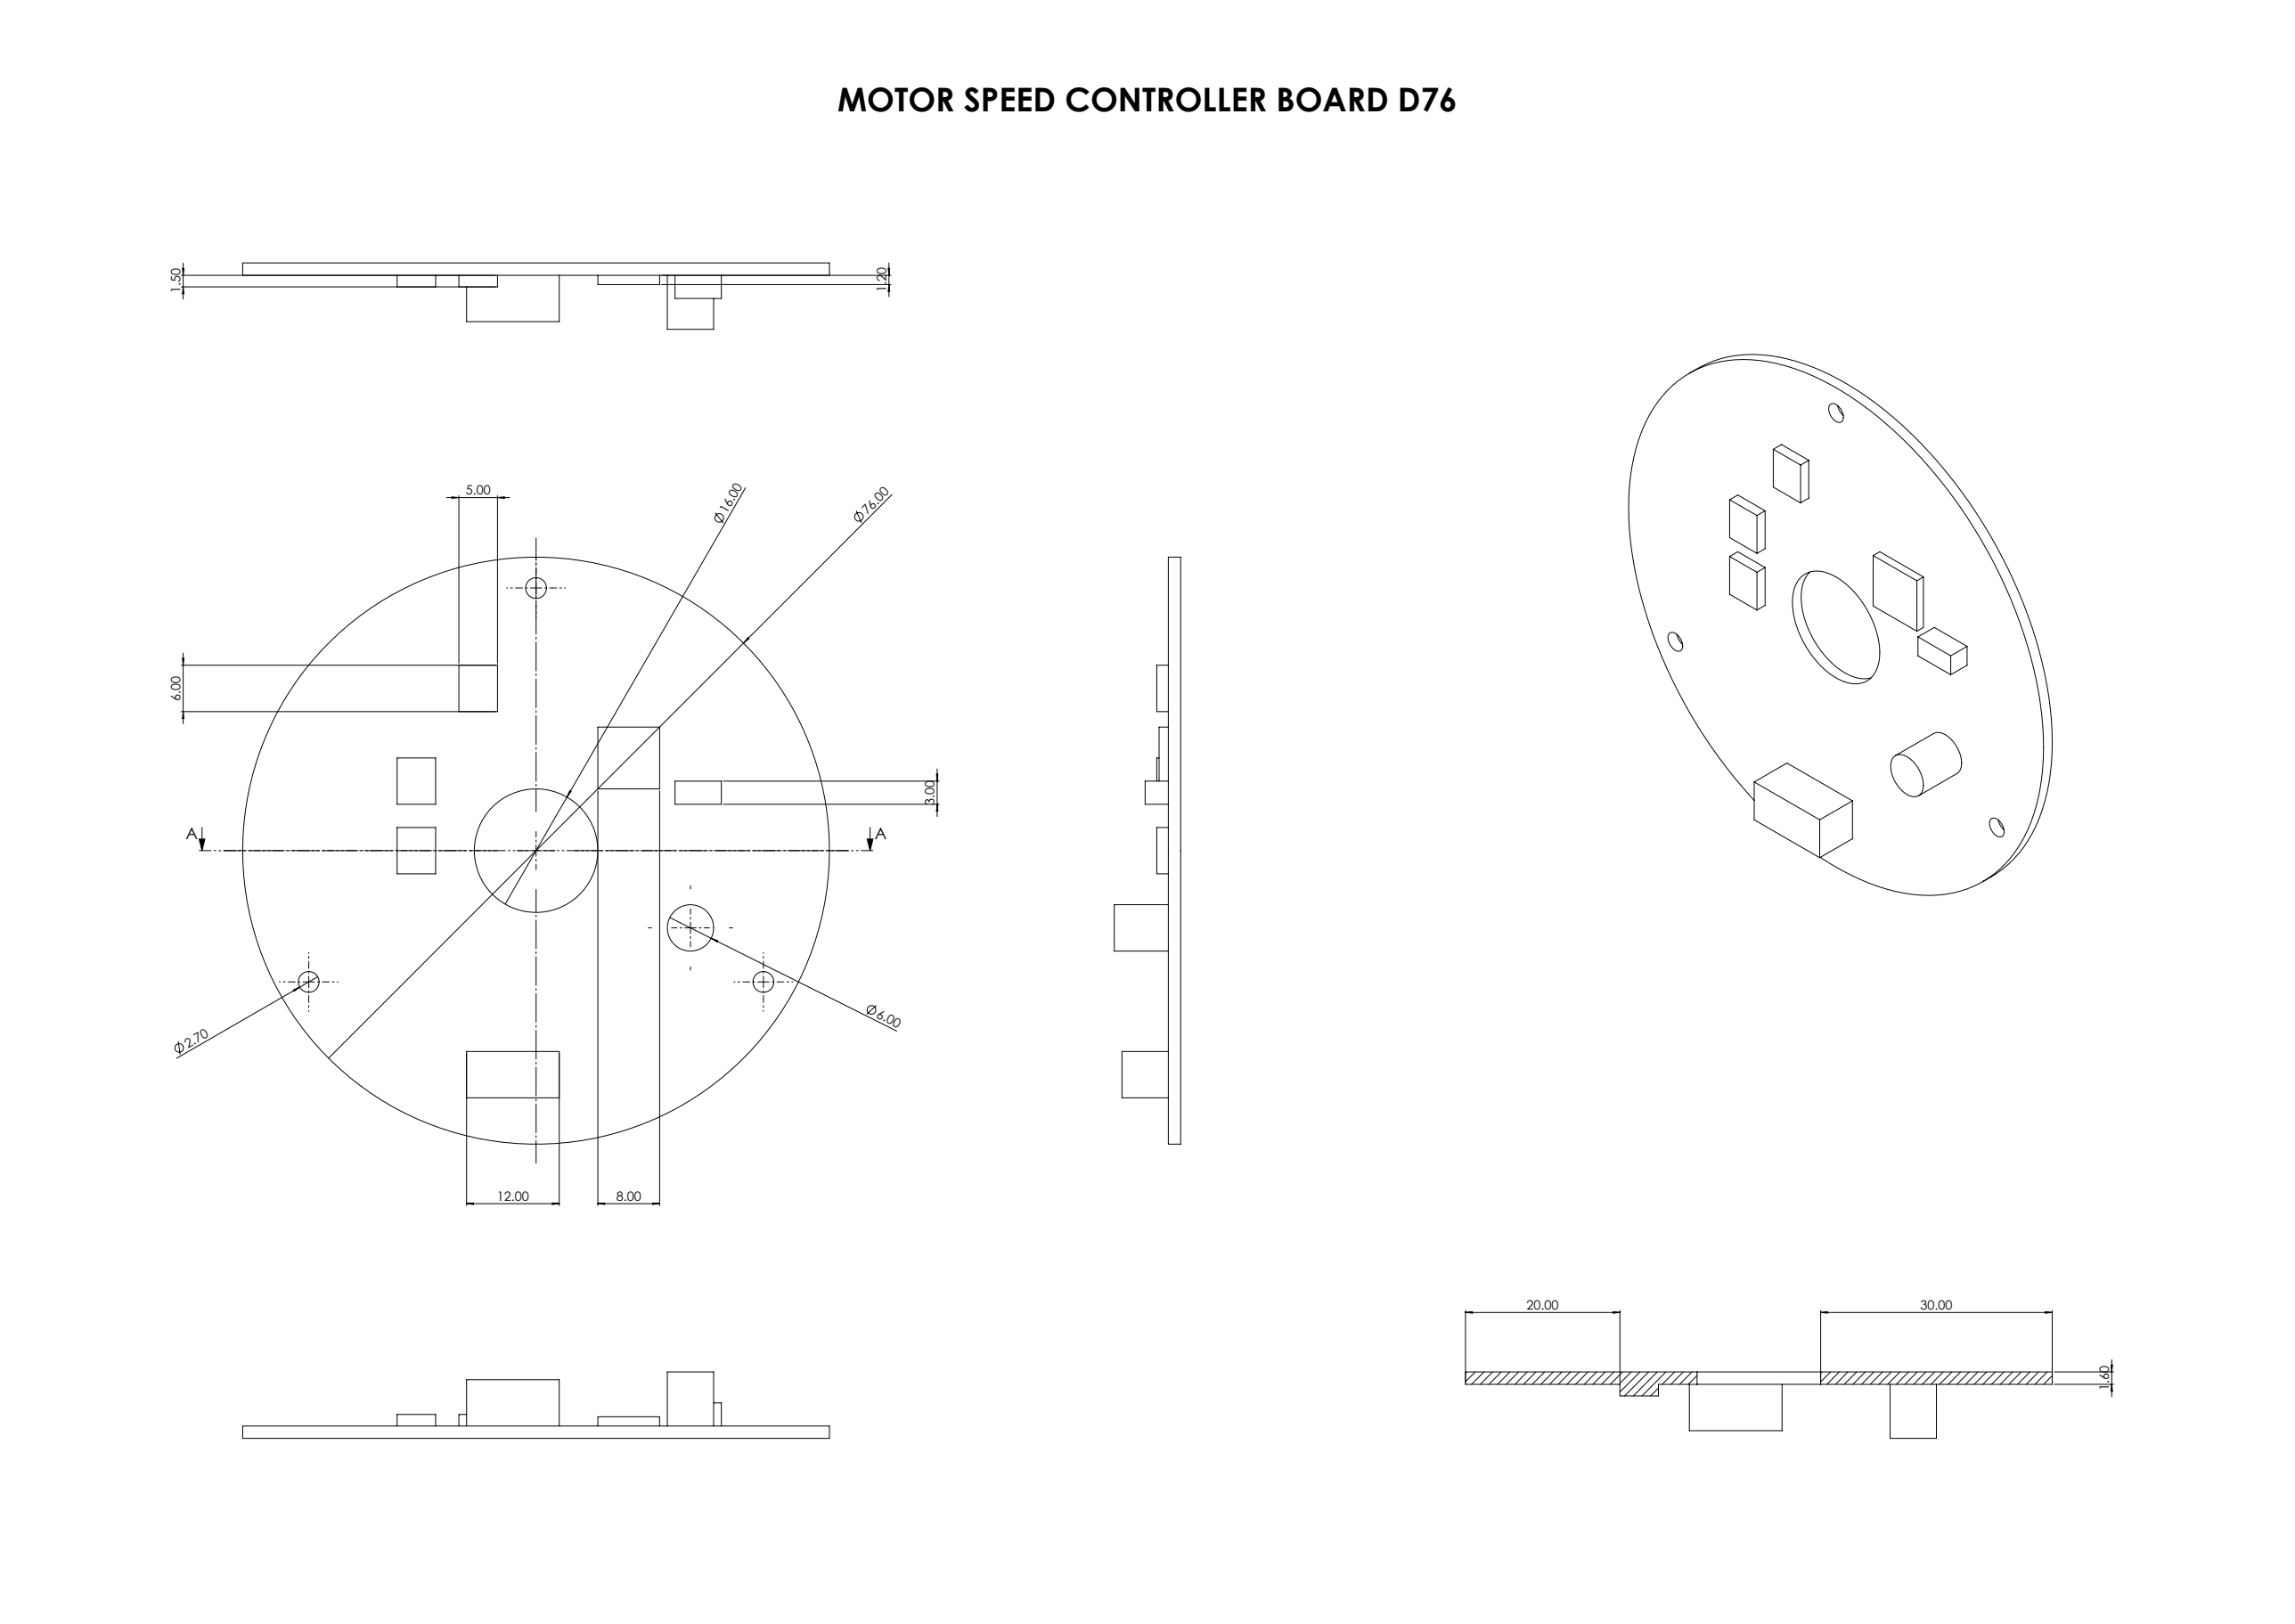
ISO-10303-21;
HEADER;
/* Generated by software containing ST-Developer
 * from STEP Tools, Inc. (www.steptools.com) 
 */

FILE_DESCRIPTION(
/* description */ (''),
/* implementation_level */ '2;1');

FILE_NAME(
/* name */ '13_Motor_Speed_Controller_Board_D76.step',
/* time_stamp */ '2026-10-19T23:00:43-07:00',
/* author */ (''),
/* organization */ (''),
/* preprocessor_version */ 'ST-DEVELOPER v20.2',
/* originating_system */ 'Autodesk Translation Framework v15.15.0.0',
/* authorisation */ '');

FILE_SCHEMA (('AUTOMOTIVE_DESIGN { 1 0 10303 214 3 1 1 }'));
ENDSEC;

DATA;
#10=MECHANICAL_DESIGN_GEOMETRIC_PRESENTATION_REPRESENTATION('',(#1008),#55002);
#968=SHAPE_REPRESENTATION_RELATIONSHIP('SRR','None',#55116,#988);
#988=ADVANCED_BREP_SHAPE_REPRESENTATION('',(#1028),#54994);
#1008=STYLED_ITEM('',(#55379),#1028);
#1028=MANIFOLD_SOLID_BREP('Controller Board',#24541);
#1244=FACE_BOUND('',#4664,.T.);
#1245=FACE_BOUND('',#4665,.T.);
#1246=FACE_BOUND('',#4666,.T.);
#1247=FACE_BOUND('',#4667,.T.);
#1248=FACE_BOUND('',#4670,.T.);
#1249=FACE_BOUND('',#4671,.T.);
#1250=FACE_BOUND('',#4672,.T.);
#1251=FACE_BOUND('',#4673,.T.);
#1252=FACE_BOUND('',#4674,.T.);
#1253=FACE_BOUND('',#4675,.T.);
#1254=FACE_BOUND('',#4676,.T.);
#1255=FACE_BOUND('',#4677,.T.);
#1256=FACE_BOUND('',#4678,.T.);
#1257=FACE_BOUND('',#4679,.T.);
#1258=FACE_BOUND('',#4680,.T.);
#1504=PLANE('',#26100);
#1505=PLANE('',#26101);
#1506=PLANE('',#26102);
#1507=PLANE('',#26103);
#1508=PLANE('',#26104);
#1509=PLANE('',#26105);
#1510=PLANE('',#26106);
#1511=PLANE('',#26107);
#1512=PLANE('',#26108);
#1513=PLANE('',#26109);
#1514=PLANE('',#26113);
#1515=PLANE('',#26114);
#1516=PLANE('',#26115);
#1517=PLANE('',#26116);
#1518=PLANE('',#26117);
#1519=PLANE('',#26118);
#1520=PLANE('',#26119);
#1521=PLANE('',#26120);
#1522=PLANE('',#26121);
#1523=PLANE('',#26122);
#1524=PLANE('',#26123);
#1525=PLANE('',#26124);
#1526=PLANE('',#26125);
#1527=PLANE('',#26126);
#1528=PLANE('',#26127);
#1529=PLANE('',#26128);
#1530=PLANE('',#26129);
#1531=PLANE('',#26130);
#1532=PLANE('',#26131);
#1533=PLANE('',#26132);
#1534=PLANE('',#26133);
#1535=PLANE('',#26146);
#1536=PLANE('',#26150);
#2187=CYLINDRICAL_SURFACE('',#26110,0.3);
#2188=CYLINDRICAL_SURFACE('',#26134,0.135);
#2189=CYLINDRICAL_SURFACE('',#26137,0.135);
#2190=CYLINDRICAL_SURFACE('',#26140,0.135);
#2191=CYLINDRICAL_SURFACE('',#26143,0.8);
#2192=CYLINDRICAL_SURFACE('',#26148,3.8);
#3055=FACE_OUTER_BOUND('',#4627,.T.);
#3056=FACE_OUTER_BOUND('',#4628,.T.);
#3057=FACE_OUTER_BOUND('',#4629,.T.);
#3058=FACE_OUTER_BOUND('',#4630,.T.);
#3059=FACE_OUTER_BOUND('',#4631,.T.);
#3060=FACE_OUTER_BOUND('',#4632,.T.);
#3061=FACE_OUTER_BOUND('',#4633,.T.);
#3062=FACE_OUTER_BOUND('',#4634,.T.);
#3063=FACE_OUTER_BOUND('',#4635,.T.);
#3064=FACE_OUTER_BOUND('',#4636,.T.);
#3065=FACE_OUTER_BOUND('',#4637,.T.);
#3066=FACE_OUTER_BOUND('',#4638,.T.);
#3067=FACE_OUTER_BOUND('',#4639,.T.);
#3068=FACE_OUTER_BOUND('',#4640,.T.);
#3069=FACE_OUTER_BOUND('',#4641,.T.);
#3070=FACE_OUTER_BOUND('',#4642,.T.);
#3071=FACE_OUTER_BOUND('',#4643,.T.);
#3072=FACE_OUTER_BOUND('',#4644,.T.);
#3073=FACE_OUTER_BOUND('',#4645,.T.);
#3074=FACE_OUTER_BOUND('',#4646,.T.);
#3075=FACE_OUTER_BOUND('',#4647,.T.);
#3076=FACE_OUTER_BOUND('',#4648,.T.);
#3077=FACE_OUTER_BOUND('',#4649,.T.);
#3078=FACE_OUTER_BOUND('',#4650,.T.);
#3079=FACE_OUTER_BOUND('',#4651,.T.);
#3080=FACE_OUTER_BOUND('',#4652,.T.);
#3081=FACE_OUTER_BOUND('',#4653,.T.);
#3082=FACE_OUTER_BOUND('',#4654,.T.);
#3083=FACE_OUTER_BOUND('',#4655,.T.);
#3084=FACE_OUTER_BOUND('',#4656,.T.);
#3085=FACE_OUTER_BOUND('',#4657,.T.);
#3086=FACE_OUTER_BOUND('',#4658,.T.);
#3087=FACE_OUTER_BOUND('',#4659,.T.);
#3088=FACE_OUTER_BOUND('',#4660,.T.);
#3089=FACE_OUTER_BOUND('',#4661,.T.);
#3090=FACE_OUTER_BOUND('',#4662,.T.);
#3091=FACE_OUTER_BOUND('',#4663,.T.);
#3092=FACE_OUTER_BOUND('',#4668,.T.);
#3093=FACE_OUTER_BOUND('',#4669,.T.);
#4627=EDGE_LOOP('',(#18894,#18895,#18896,#18897));
#4628=EDGE_LOOP('',(#18898,#18899,#18900,#18901));
#4629=EDGE_LOOP('',(#18902,#18903,#18904,#18905));
#4630=EDGE_LOOP('',(#18906,#18907,#18908,#18909));
#4631=EDGE_LOOP('',(#18910,#18911,#18912,#18913));
#4632=EDGE_LOOP('',(#18914,#18915,#18916,#18917));
#4633=EDGE_LOOP('',(#18918,#18919,#18920,#18921));
#4634=EDGE_LOOP('',(#18922,#18923,#18924,#18925));
#4635=EDGE_LOOP('',(#18926,#18927,#18928,#18929));
#4636=EDGE_LOOP('',(#18930,#18931,#18932,#18933));
#4637=EDGE_LOOP('',(#18934,#18935,#18936,#18937));
#4638=EDGE_LOOP('',(#18938));
#4639=EDGE_LOOP('',(#18939,#18940,#18941,#18942));
#4640=EDGE_LOOP('',(#18943,#18944,#18945,#18946));
#4641=EDGE_LOOP('',(#18947,#18948,#18949,#18950));
#4642=EDGE_LOOP('',(#18951,#18952,#18953,#18954));
#4643=EDGE_LOOP('',(#18955,#18956,#18957,#18958));
#4644=EDGE_LOOP('',(#18959,#18960,#18961,#18962));
#4645=EDGE_LOOP('',(#18963,#18964,#18965,#18966));
#4646=EDGE_LOOP('',(#18967,#18968,#18969,#18970));
#4647=EDGE_LOOP('',(#18971,#18972,#18973,#18974));
#4648=EDGE_LOOP('',(#18975,#18976,#18977,#18978));
#4649=EDGE_LOOP('',(#18979,#18980,#18981,#18982));
#4650=EDGE_LOOP('',(#18983,#18984,#18985,#18986));
#4651=EDGE_LOOP('',(#18987,#18988,#18989,#18990));
#4652=EDGE_LOOP('',(#18991,#18992,#18993,#18994));
#4653=EDGE_LOOP('',(#18995,#18996,#18997,#18998));
#4654=EDGE_LOOP('',(#18999,#19000,#19001,#19002));
#4655=EDGE_LOOP('',(#19003,#19004,#19005,#19006));
#4656=EDGE_LOOP('',(#19007,#19008,#19009,#19010));
#4657=EDGE_LOOP('',(#19011,#19012,#19013,#19014));
#4658=EDGE_LOOP('',(#19015,#19016,#19017,#19018));
#4659=EDGE_LOOP('',(#19019,#19020,#19021,#19022));
#4660=EDGE_LOOP('',(#19023,#19024,#19025,#19026));
#4661=EDGE_LOOP('',(#19027,#19028,#19029,#19030));
#4662=EDGE_LOOP('',(#19031,#19032,#19033,#19034));
#4663=EDGE_LOOP('',(#19035));
#4664=EDGE_LOOP('',(#19036));
#4665=EDGE_LOOP('',(#19037));
#4666=EDGE_LOOP('',(#19038));
#4667=EDGE_LOOP('',(#19039));
#4668=EDGE_LOOP('',(#19040,#19041,#19042,#19043));
#4669=EDGE_LOOP('',(#19044));
#4670=EDGE_LOOP('',(#19045,#19046,#19047,#19048));
#4671=EDGE_LOOP('',(#19049,#19050,#19051,#19052));
#4672=EDGE_LOOP('',(#19053,#19054,#19055,#19056));
#4673=EDGE_LOOP('',(#19057,#19058,#19059,#19060));
#4674=EDGE_LOOP('',(#19061,#19062,#19063,#19064));
#4675=EDGE_LOOP('',(#19065));
#4676=EDGE_LOOP('',(#19066));
#4677=EDGE_LOOP('',(#19067));
#4678=EDGE_LOOP('',(#19068));
#4679=EDGE_LOOP('',(#19069));
#4680=EDGE_LOOP('',(#19070,#19071,#19072,#19073));
#6187=LINE('',#37562,#8008);
#6188=LINE('',#37564,#8009);
#6189=LINE('',#37566,#8010);
#6190=LINE('',#37567,#8011);
#6191=LINE('',#37570,#8012);
#6192=LINE('',#37572,#8013);
#6193=LINE('',#37573,#8014);
#6194=LINE('',#37576,#8015);
#6195=LINE('',#37578,#8016);
#6196=LINE('',#37579,#8017);
#6197=LINE('',#37581,#8018);
#6198=LINE('',#37582,#8019);
#6199=LINE('',#37587,#8020);
#6200=LINE('',#37589,#8021);
#6201=LINE('',#37591,#8022);
#6202=LINE('',#37592,#8023);
#6203=LINE('',#37595,#8024);
#6204=LINE('',#37597,#8025);
#6205=LINE('',#37598,#8026);
#6206=LINE('',#37601,#8027);
#6207=LINE('',#37603,#8028);
#6208=LINE('',#37604,#8029);
#6209=LINE('',#37606,#8030);
#6210=LINE('',#37607,#8031);
#6211=LINE('',#37613,#8032);
#6212=LINE('',#37619,#8033);
#6213=LINE('',#37621,#8034);
#6214=LINE('',#37623,#8035);
#6215=LINE('',#37624,#8036);
#6216=LINE('',#37627,#8037);
#6217=LINE('',#37629,#8038);
#6218=LINE('',#37630,#8039);
#6219=LINE('',#37633,#8040);
#6220=LINE('',#37635,#8041);
#6221=LINE('',#37636,#8042);
#6222=LINE('',#37638,#8043);
#6223=LINE('',#37639,#8044);
#6224=LINE('',#37644,#8045);
#6225=LINE('',#37646,#8046);
#6226=LINE('',#37648,#8047);
#6227=LINE('',#37649,#8048);
#6228=LINE('',#37652,#8049);
#6229=LINE('',#37654,#8050);
#6230=LINE('',#37655,#8051);
#6231=LINE('',#37658,#8052);
#6232=LINE('',#37660,#8053);
#6233=LINE('',#37661,#8054);
#6234=LINE('',#37663,#8055);
#6235=LINE('',#37664,#8056);
#6236=LINE('',#37669,#8057);
#6237=LINE('',#37671,#8058);
#6238=LINE('',#37673,#8059);
#6239=LINE('',#37674,#8060);
#6240=LINE('',#37677,#8061);
#6241=LINE('',#37679,#8062);
#6242=LINE('',#37680,#8063);
#6243=LINE('',#37683,#8064);
#6244=LINE('',#37685,#8065);
#6245=LINE('',#37686,#8066);
#6246=LINE('',#37688,#8067);
#6247=LINE('',#37689,#8068);
#6248=LINE('',#37694,#8069);
#6249=LINE('',#37696,#8070);
#6250=LINE('',#37698,#8071);
#6251=LINE('',#37699,#8072);
#6252=LINE('',#37702,#8073);
#6253=LINE('',#37704,#8074);
#6254=LINE('',#37705,#8075);
#6255=LINE('',#37708,#8076);
#6256=LINE('',#37710,#8077);
#6257=LINE('',#37711,#8078);
#6258=LINE('',#37713,#8079);
#6259=LINE('',#37714,#8080);
#6260=LINE('',#37720,#8081);
#6261=LINE('',#37726,#8082);
#6262=LINE('',#37732,#8083);
#6263=LINE('',#37738,#8084);
#6264=LINE('',#37746,#8085);
#8008=VECTOR('',#30665,1.);
#8009=VECTOR('',#30666,1.);
#8010=VECTOR('',#30667,1.);
#8011=VECTOR('',#30668,1.);
#8012=VECTOR('',#30671,1.);
#8013=VECTOR('',#30672,1.);
#8014=VECTOR('',#30673,1.);
#8015=VECTOR('',#30676,1.);
#8016=VECTOR('',#30677,1.);
#8017=VECTOR('',#30678,1.);
#8018=VECTOR('',#30681,1.);
#8019=VECTOR('',#30682,1.);
#8020=VECTOR('',#30687,1.);
#8021=VECTOR('',#30688,1.);
#8022=VECTOR('',#30689,1.);
#8023=VECTOR('',#30690,1.);
#8024=VECTOR('',#30693,1.);
#8025=VECTOR('',#30694,1.);
#8026=VECTOR('',#30695,1.);
#8027=VECTOR('',#30698,1.);
#8028=VECTOR('',#30699,1.);
#8029=VECTOR('',#30700,1.);
#8030=VECTOR('',#30703,1.);
#8031=VECTOR('',#30704,1.);
#8032=VECTOR('',#30711,0.3);
#8033=VECTOR('',#30718,1.);
#8034=VECTOR('',#30719,1.);
#8035=VECTOR('',#30720,1.);
#8036=VECTOR('',#30721,1.);
#8037=VECTOR('',#30724,1.);
#8038=VECTOR('',#30725,1.);
#8039=VECTOR('',#30726,1.);
#8040=VECTOR('',#30729,1.);
#8041=VECTOR('',#30730,1.);
#8042=VECTOR('',#30731,1.);
#8043=VECTOR('',#30734,1.);
#8044=VECTOR('',#30735,1.);
#8045=VECTOR('',#30740,1.);
#8046=VECTOR('',#30741,1.);
#8047=VECTOR('',#30742,1.);
#8048=VECTOR('',#30743,1.);
#8049=VECTOR('',#30746,1.);
#8050=VECTOR('',#30747,1.);
#8051=VECTOR('',#30748,1.);
#8052=VECTOR('',#30751,1.);
#8053=VECTOR('',#30752,1.);
#8054=VECTOR('',#30753,1.);
#8055=VECTOR('',#30756,1.);
#8056=VECTOR('',#30757,1.);
#8057=VECTOR('',#30762,1.);
#8058=VECTOR('',#30763,1.);
#8059=VECTOR('',#30764,1.);
#8060=VECTOR('',#30765,1.);
#8061=VECTOR('',#30768,1.);
#8062=VECTOR('',#30769,1.);
#8063=VECTOR('',#30770,1.);
#8064=VECTOR('',#30773,1.);
#8065=VECTOR('',#30774,1.);
#8066=VECTOR('',#30775,1.);
#8067=VECTOR('',#30778,1.);
#8068=VECTOR('',#30779,1.);
#8069=VECTOR('',#30784,1.);
#8070=VECTOR('',#30785,1.);
#8071=VECTOR('',#30786,1.);
#8072=VECTOR('',#30787,1.);
#8073=VECTOR('',#30790,1.);
#8074=VECTOR('',#30791,1.);
#8075=VECTOR('',#30792,1.);
#8076=VECTOR('',#30795,1.);
#8077=VECTOR('',#30796,1.);
#8078=VECTOR('',#30797,1.);
#8079=VECTOR('',#30800,1.);
#8080=VECTOR('',#30801,1.);
#8081=VECTOR('',#30808,0.135);
#8082=VECTOR('',#30815,0.135);
#8083=VECTOR('',#30822,0.135);
#8084=VECTOR('',#30829,0.8);
#8085=VECTOR('',#30840,3.8);
#9698=CIRCLE('',#26111,0.3);
#9699=CIRCLE('',#26112,0.3);
#9700=CIRCLE('',#26135,0.135);
#9701=CIRCLE('',#26136,0.135);
#9702=CIRCLE('',#26138,0.135);
#9703=CIRCLE('',#26139,0.135);
#9704=CIRCLE('',#26141,0.135);
#9705=CIRCLE('',#26142,0.135);
#9706=CIRCLE('',#26144,0.8);
#9707=CIRCLE('',#26145,0.8);
#9708=CIRCLE('',#26147,3.8);
#9709=CIRCLE('',#26149,3.8);
#11001=VERTEX_POINT('',#37560);
#11002=VERTEX_POINT('',#37561);
#11003=VERTEX_POINT('',#37563);
#11004=VERTEX_POINT('',#37565);
#11005=VERTEX_POINT('',#37569);
#11006=VERTEX_POINT('',#37571);
#11007=VERTEX_POINT('',#37575);
#11008=VERTEX_POINT('',#37577);
#11009=VERTEX_POINT('',#37585);
#11010=VERTEX_POINT('',#37586);
#11011=VERTEX_POINT('',#37588);
#11012=VERTEX_POINT('',#37590);
#11013=VERTEX_POINT('',#37594);
#11014=VERTEX_POINT('',#37596);
#11015=VERTEX_POINT('',#37600);
#11016=VERTEX_POINT('',#37602);
#11017=VERTEX_POINT('',#37610);
#11018=VERTEX_POINT('',#37612);
#11019=VERTEX_POINT('',#37617);
#11020=VERTEX_POINT('',#37618);
#11021=VERTEX_POINT('',#37620);
#11022=VERTEX_POINT('',#37622);
#11023=VERTEX_POINT('',#37626);
#11024=VERTEX_POINT('',#37628);
#11025=VERTEX_POINT('',#37632);
#11026=VERTEX_POINT('',#37634);
#11027=VERTEX_POINT('',#37642);
#11028=VERTEX_POINT('',#37643);
#11029=VERTEX_POINT('',#37645);
#11030=VERTEX_POINT('',#37647);
#11031=VERTEX_POINT('',#37651);
#11032=VERTEX_POINT('',#37653);
#11033=VERTEX_POINT('',#37657);
#11034=VERTEX_POINT('',#37659);
#11035=VERTEX_POINT('',#37667);
#11036=VERTEX_POINT('',#37668);
#11037=VERTEX_POINT('',#37670);
#11038=VERTEX_POINT('',#37672);
#11039=VERTEX_POINT('',#37676);
#11040=VERTEX_POINT('',#37678);
#11041=VERTEX_POINT('',#37682);
#11042=VERTEX_POINT('',#37684);
#11043=VERTEX_POINT('',#37692);
#11044=VERTEX_POINT('',#37693);
#11045=VERTEX_POINT('',#37695);
#11046=VERTEX_POINT('',#37697);
#11047=VERTEX_POINT('',#37701);
#11048=VERTEX_POINT('',#37703);
#11049=VERTEX_POINT('',#37707);
#11050=VERTEX_POINT('',#37709);
#11051=VERTEX_POINT('',#37717);
#11052=VERTEX_POINT('',#37719);
#11053=VERTEX_POINT('',#37723);
#11054=VERTEX_POINT('',#37725);
#11055=VERTEX_POINT('',#37729);
#11056=VERTEX_POINT('',#37731);
#11057=VERTEX_POINT('',#37735);
#11058=VERTEX_POINT('',#37737);
#11059=VERTEX_POINT('',#37741);
#11060=VERTEX_POINT('',#37744);
#13855=EDGE_CURVE('',#11001,#11002,#6187,.T.);
#13856=EDGE_CURVE('',#11001,#11003,#6188,.T.);
#13857=EDGE_CURVE('',#11004,#11003,#6189,.T.);
#13858=EDGE_CURVE('',#11002,#11004,#6190,.T.);
#13859=EDGE_CURVE('',#11002,#11005,#6191,.T.);
#13860=EDGE_CURVE('',#11006,#11004,#6192,.T.);
#13861=EDGE_CURVE('',#11005,#11006,#6193,.T.);
#13862=EDGE_CURVE('',#11005,#11007,#6194,.T.);
#13863=EDGE_CURVE('',#11008,#11006,#6195,.T.);
#13864=EDGE_CURVE('',#11007,#11008,#6196,.T.);
#13865=EDGE_CURVE('',#11007,#11001,#6197,.T.);
#13866=EDGE_CURVE('',#11003,#11008,#6198,.T.);
#13867=EDGE_CURVE('',#11009,#11010,#6199,.T.);
#13868=EDGE_CURVE('',#11009,#11011,#6200,.T.);
#13869=EDGE_CURVE('',#11012,#11011,#6201,.T.);
#13870=EDGE_CURVE('',#11010,#11012,#6202,.T.);
#13871=EDGE_CURVE('',#11010,#11013,#6203,.T.);
#13872=EDGE_CURVE('',#11014,#11012,#6204,.T.);
#13873=EDGE_CURVE('',#11013,#11014,#6205,.T.);
#13874=EDGE_CURVE('',#11013,#11015,#6206,.T.);
#13875=EDGE_CURVE('',#11016,#11014,#6207,.T.);
#13876=EDGE_CURVE('',#11015,#11016,#6208,.T.);
#13877=EDGE_CURVE('',#11015,#11009,#6209,.T.);
#13878=EDGE_CURVE('',#11011,#11016,#6210,.T.);
#13879=EDGE_CURVE('',#11017,#11017,#9698,.T.);
#13880=EDGE_CURVE('',#11017,#11018,#6211,.T.);
#13881=EDGE_CURVE('',#11018,#11018,#9699,.T.);
#13882=EDGE_CURVE('',#11019,#11020,#6212,.T.);
#13883=EDGE_CURVE('',#11019,#11021,#6213,.T.);
#13884=EDGE_CURVE('',#11022,#11021,#6214,.T.);
#13885=EDGE_CURVE('',#11020,#11022,#6215,.T.);
#13886=EDGE_CURVE('',#11020,#11023,#6216,.T.);
#13887=EDGE_CURVE('',#11024,#11022,#6217,.T.);
#13888=EDGE_CURVE('',#11023,#11024,#6218,.T.);
#13889=EDGE_CURVE('',#11023,#11025,#6219,.T.);
#13890=EDGE_CURVE('',#11026,#11024,#6220,.T.);
#13891=EDGE_CURVE('',#11025,#11026,#6221,.T.);
#13892=EDGE_CURVE('',#11025,#11019,#6222,.T.);
#13893=EDGE_CURVE('',#11021,#11026,#6223,.T.);
#13894=EDGE_CURVE('',#11027,#11028,#6224,.T.);
#13895=EDGE_CURVE('',#11027,#11029,#6225,.T.);
#13896=EDGE_CURVE('',#11030,#11029,#6226,.T.);
#13897=EDGE_CURVE('',#11028,#11030,#6227,.T.);
#13898=EDGE_CURVE('',#11028,#11031,#6228,.T.);
#13899=EDGE_CURVE('',#11032,#11030,#6229,.T.);
#13900=EDGE_CURVE('',#11031,#11032,#6230,.T.);
#13901=EDGE_CURVE('',#11031,#11033,#6231,.T.);
#13902=EDGE_CURVE('',#11034,#11032,#6232,.T.);
#13903=EDGE_CURVE('',#11033,#11034,#6233,.T.);
#13904=EDGE_CURVE('',#11033,#11027,#6234,.T.);
#13905=EDGE_CURVE('',#11029,#11034,#6235,.T.);
#13906=EDGE_CURVE('',#11035,#11036,#6236,.T.);
#13907=EDGE_CURVE('',#11035,#11037,#6237,.T.);
#13908=EDGE_CURVE('',#11038,#11037,#6238,.T.);
#13909=EDGE_CURVE('',#11036,#11038,#6239,.T.);
#13910=EDGE_CURVE('',#11036,#11039,#6240,.T.);
#13911=EDGE_CURVE('',#11040,#11038,#6241,.T.);
#13912=EDGE_CURVE('',#11039,#11040,#6242,.T.);
#13913=EDGE_CURVE('',#11039,#11041,#6243,.T.);
#13914=EDGE_CURVE('',#11042,#11040,#6244,.T.);
#13915=EDGE_CURVE('',#11041,#11042,#6245,.T.);
#13916=EDGE_CURVE('',#11041,#11035,#6246,.T.);
#13917=EDGE_CURVE('',#11037,#11042,#6247,.T.);
#13918=EDGE_CURVE('',#11043,#11044,#6248,.T.);
#13919=EDGE_CURVE('',#11043,#11045,#6249,.T.);
#13920=EDGE_CURVE('',#11046,#11045,#6250,.T.);
#13921=EDGE_CURVE('',#11044,#11046,#6251,.T.);
#13922=EDGE_CURVE('',#11044,#11047,#6252,.T.);
#13923=EDGE_CURVE('',#11048,#11046,#6253,.T.);
#13924=EDGE_CURVE('',#11047,#11048,#6254,.T.);
#13925=EDGE_CURVE('',#11047,#11049,#6255,.T.);
#13926=EDGE_CURVE('',#11050,#11048,#6256,.T.);
#13927=EDGE_CURVE('',#11049,#11050,#6257,.T.);
#13928=EDGE_CURVE('',#11049,#11043,#6258,.T.);
#13929=EDGE_CURVE('',#11045,#11050,#6259,.T.);
#13930=EDGE_CURVE('',#11051,#11051,#9700,.T.);
#13931=EDGE_CURVE('',#11051,#11052,#6260,.T.);
#13932=EDGE_CURVE('',#11052,#11052,#9701,.T.);
#13933=EDGE_CURVE('',#11053,#11053,#9702,.T.);
#13934=EDGE_CURVE('',#11053,#11054,#6261,.T.);
#13935=EDGE_CURVE('',#11054,#11054,#9703,.T.);
#13936=EDGE_CURVE('',#11055,#11055,#9704,.T.);
#13937=EDGE_CURVE('',#11055,#11056,#6262,.T.);
#13938=EDGE_CURVE('',#11056,#11056,#9705,.T.);
#13939=EDGE_CURVE('',#11057,#11057,#9706,.T.);
#13940=EDGE_CURVE('',#11057,#11058,#6263,.T.);
#13941=EDGE_CURVE('',#11058,#11058,#9707,.T.);
#13942=EDGE_CURVE('',#11059,#11059,#9708,.T.);
#13943=EDGE_CURVE('',#11060,#11060,#9709,.T.);
#13944=EDGE_CURVE('',#11060,#11059,#6264,.T.);
#18894=ORIENTED_EDGE('',*,*,#13855,.F.);
#18895=ORIENTED_EDGE('',*,*,#13856,.T.);
#18896=ORIENTED_EDGE('',*,*,#13857,.F.);
#18897=ORIENTED_EDGE('',*,*,#13858,.F.);
#18898=ORIENTED_EDGE('',*,*,#13859,.F.);
#18899=ORIENTED_EDGE('',*,*,#13858,.T.);
#18900=ORIENTED_EDGE('',*,*,#13860,.F.);
#18901=ORIENTED_EDGE('',*,*,#13861,.F.);
#18902=ORIENTED_EDGE('',*,*,#13862,.F.);
#18903=ORIENTED_EDGE('',*,*,#13861,.T.);
#18904=ORIENTED_EDGE('',*,*,#13863,.F.);
#18905=ORIENTED_EDGE('',*,*,#13864,.F.);
#18906=ORIENTED_EDGE('',*,*,#13865,.F.);
#18907=ORIENTED_EDGE('',*,*,#13864,.T.);
#18908=ORIENTED_EDGE('',*,*,#13866,.F.);
#18909=ORIENTED_EDGE('',*,*,#13856,.F.);
#18910=ORIENTED_EDGE('',*,*,#13866,.T.);
#18911=ORIENTED_EDGE('',*,*,#13863,.T.);
#18912=ORIENTED_EDGE('',*,*,#13860,.T.);
#18913=ORIENTED_EDGE('',*,*,#13857,.T.);
#18914=ORIENTED_EDGE('',*,*,#13867,.F.);
#18915=ORIENTED_EDGE('',*,*,#13868,.T.);
#18916=ORIENTED_EDGE('',*,*,#13869,.F.);
#18917=ORIENTED_EDGE('',*,*,#13870,.F.);
#18918=ORIENTED_EDGE('',*,*,#13871,.F.);
#18919=ORIENTED_EDGE('',*,*,#13870,.T.);
#18920=ORIENTED_EDGE('',*,*,#13872,.F.);
#18921=ORIENTED_EDGE('',*,*,#13873,.F.);
#18922=ORIENTED_EDGE('',*,*,#13874,.F.);
#18923=ORIENTED_EDGE('',*,*,#13873,.T.);
#18924=ORIENTED_EDGE('',*,*,#13875,.F.);
#18925=ORIENTED_EDGE('',*,*,#13876,.F.);
#18926=ORIENTED_EDGE('',*,*,#13877,.F.);
#18927=ORIENTED_EDGE('',*,*,#13876,.T.);
#18928=ORIENTED_EDGE('',*,*,#13878,.F.);
#18929=ORIENTED_EDGE('',*,*,#13868,.F.);
#18930=ORIENTED_EDGE('',*,*,#13878,.T.);
#18931=ORIENTED_EDGE('',*,*,#13875,.T.);
#18932=ORIENTED_EDGE('',*,*,#13872,.T.);
#18933=ORIENTED_EDGE('',*,*,#13869,.T.);
#18934=ORIENTED_EDGE('',*,*,#13879,.F.);
#18935=ORIENTED_EDGE('',*,*,#13880,.T.);
#18936=ORIENTED_EDGE('',*,*,#13881,.F.);
#18937=ORIENTED_EDGE('',*,*,#13880,.F.);
#18938=ORIENTED_EDGE('',*,*,#13879,.T.);
#18939=ORIENTED_EDGE('',*,*,#13882,.F.);
#18940=ORIENTED_EDGE('',*,*,#13883,.T.);
#18941=ORIENTED_EDGE('',*,*,#13884,.F.);
#18942=ORIENTED_EDGE('',*,*,#13885,.F.);
#18943=ORIENTED_EDGE('',*,*,#13886,.F.);
#18944=ORIENTED_EDGE('',*,*,#13885,.T.);
#18945=ORIENTED_EDGE('',*,*,#13887,.F.);
#18946=ORIENTED_EDGE('',*,*,#13888,.F.);
#18947=ORIENTED_EDGE('',*,*,#13889,.F.);
#18948=ORIENTED_EDGE('',*,*,#13888,.T.);
#18949=ORIENTED_EDGE('',*,*,#13890,.F.);
#18950=ORIENTED_EDGE('',*,*,#13891,.F.);
#18951=ORIENTED_EDGE('',*,*,#13892,.F.);
#18952=ORIENTED_EDGE('',*,*,#13891,.T.);
#18953=ORIENTED_EDGE('',*,*,#13893,.F.);
#18954=ORIENTED_EDGE('',*,*,#13883,.F.);
#18955=ORIENTED_EDGE('',*,*,#13893,.T.);
#18956=ORIENTED_EDGE('',*,*,#13890,.T.);
#18957=ORIENTED_EDGE('',*,*,#13887,.T.);
#18958=ORIENTED_EDGE('',*,*,#13884,.T.);
#18959=ORIENTED_EDGE('',*,*,#13894,.F.);
#18960=ORIENTED_EDGE('',*,*,#13895,.T.);
#18961=ORIENTED_EDGE('',*,*,#13896,.F.);
#18962=ORIENTED_EDGE('',*,*,#13897,.F.);
#18963=ORIENTED_EDGE('',*,*,#13898,.F.);
#18964=ORIENTED_EDGE('',*,*,#13897,.T.);
#18965=ORIENTED_EDGE('',*,*,#13899,.F.);
#18966=ORIENTED_EDGE('',*,*,#13900,.F.);
#18967=ORIENTED_EDGE('',*,*,#13901,.F.);
#18968=ORIENTED_EDGE('',*,*,#13900,.T.);
#18969=ORIENTED_EDGE('',*,*,#13902,.F.);
#18970=ORIENTED_EDGE('',*,*,#13903,.F.);
#18971=ORIENTED_EDGE('',*,*,#13904,.F.);
#18972=ORIENTED_EDGE('',*,*,#13903,.T.);
#18973=ORIENTED_EDGE('',*,*,#13905,.F.);
#18974=ORIENTED_EDGE('',*,*,#13895,.F.);
#18975=ORIENTED_EDGE('',*,*,#13905,.T.);
#18976=ORIENTED_EDGE('',*,*,#13902,.T.);
#18977=ORIENTED_EDGE('',*,*,#13899,.T.);
#18978=ORIENTED_EDGE('',*,*,#13896,.T.);
#18979=ORIENTED_EDGE('',*,*,#13906,.F.);
#18980=ORIENTED_EDGE('',*,*,#13907,.T.);
#18981=ORIENTED_EDGE('',*,*,#13908,.F.);
#18982=ORIENTED_EDGE('',*,*,#13909,.F.);
#18983=ORIENTED_EDGE('',*,*,#13910,.F.);
#18984=ORIENTED_EDGE('',*,*,#13909,.T.);
#18985=ORIENTED_EDGE('',*,*,#13911,.F.);
#18986=ORIENTED_EDGE('',*,*,#13912,.F.);
#18987=ORIENTED_EDGE('',*,*,#13913,.F.);
#18988=ORIENTED_EDGE('',*,*,#13912,.T.);
#18989=ORIENTED_EDGE('',*,*,#13914,.F.);
#18990=ORIENTED_EDGE('',*,*,#13915,.F.);
#18991=ORIENTED_EDGE('',*,*,#13916,.F.);
#18992=ORIENTED_EDGE('',*,*,#13915,.T.);
#18993=ORIENTED_EDGE('',*,*,#13917,.F.);
#18994=ORIENTED_EDGE('',*,*,#13907,.F.);
#18995=ORIENTED_EDGE('',*,*,#13917,.T.);
#18996=ORIENTED_EDGE('',*,*,#13914,.T.);
#18997=ORIENTED_EDGE('',*,*,#13911,.T.);
#18998=ORIENTED_EDGE('',*,*,#13908,.T.);
#18999=ORIENTED_EDGE('',*,*,#13918,.F.);
#19000=ORIENTED_EDGE('',*,*,#13919,.T.);
#19001=ORIENTED_EDGE('',*,*,#13920,.F.);
#19002=ORIENTED_EDGE('',*,*,#13921,.F.);
#19003=ORIENTED_EDGE('',*,*,#13922,.F.);
#19004=ORIENTED_EDGE('',*,*,#13921,.T.);
#19005=ORIENTED_EDGE('',*,*,#13923,.F.);
#19006=ORIENTED_EDGE('',*,*,#13924,.F.);
#19007=ORIENTED_EDGE('',*,*,#13925,.F.);
#19008=ORIENTED_EDGE('',*,*,#13924,.T.);
#19009=ORIENTED_EDGE('',*,*,#13926,.F.);
#19010=ORIENTED_EDGE('',*,*,#13927,.F.);
#19011=ORIENTED_EDGE('',*,*,#13928,.F.);
#19012=ORIENTED_EDGE('',*,*,#13927,.T.);
#19013=ORIENTED_EDGE('',*,*,#13929,.F.);
#19014=ORIENTED_EDGE('',*,*,#13919,.F.);
#19015=ORIENTED_EDGE('',*,*,#13929,.T.);
#19016=ORIENTED_EDGE('',*,*,#13926,.T.);
#19017=ORIENTED_EDGE('',*,*,#13923,.T.);
#19018=ORIENTED_EDGE('',*,*,#13920,.T.);
#19019=ORIENTED_EDGE('',*,*,#13930,.F.);
#19020=ORIENTED_EDGE('',*,*,#13931,.T.);
#19021=ORIENTED_EDGE('',*,*,#13932,.F.);
#19022=ORIENTED_EDGE('',*,*,#13931,.F.);
#19023=ORIENTED_EDGE('',*,*,#13933,.F.);
#19024=ORIENTED_EDGE('',*,*,#13934,.T.);
#19025=ORIENTED_EDGE('',*,*,#13935,.F.);
#19026=ORIENTED_EDGE('',*,*,#13934,.F.);
#19027=ORIENTED_EDGE('',*,*,#13936,.F.);
#19028=ORIENTED_EDGE('',*,*,#13937,.T.);
#19029=ORIENTED_EDGE('',*,*,#13938,.F.);
#19030=ORIENTED_EDGE('',*,*,#13937,.F.);
#19031=ORIENTED_EDGE('',*,*,#13939,.T.);
#19032=ORIENTED_EDGE('',*,*,#13940,.T.);
#19033=ORIENTED_EDGE('',*,*,#13941,.F.);
#19034=ORIENTED_EDGE('',*,*,#13940,.F.);
#19035=ORIENTED_EDGE('',*,*,#13942,.F.);
#19036=ORIENTED_EDGE('',*,*,#13930,.T.);
#19037=ORIENTED_EDGE('',*,*,#13933,.T.);
#19038=ORIENTED_EDGE('',*,*,#13936,.T.);
#19039=ORIENTED_EDGE('',*,*,#13941,.T.);
#19040=ORIENTED_EDGE('',*,*,#13943,.F.);
#19041=ORIENTED_EDGE('',*,*,#13944,.T.);
#19042=ORIENTED_EDGE('',*,*,#13942,.T.);
#19043=ORIENTED_EDGE('',*,*,#13944,.F.);
#19044=ORIENTED_EDGE('',*,*,#13943,.T.);
#19045=ORIENTED_EDGE('',*,*,#13867,.T.);
#19046=ORIENTED_EDGE('',*,*,#13871,.T.);
#19047=ORIENTED_EDGE('',*,*,#13874,.T.);
#19048=ORIENTED_EDGE('',*,*,#13877,.T.);
#19049=ORIENTED_EDGE('',*,*,#13882,.T.);
#19050=ORIENTED_EDGE('',*,*,#13886,.T.);
#19051=ORIENTED_EDGE('',*,*,#13889,.T.);
#19052=ORIENTED_EDGE('',*,*,#13892,.T.);
#19053=ORIENTED_EDGE('',*,*,#13894,.T.);
#19054=ORIENTED_EDGE('',*,*,#13898,.T.);
#19055=ORIENTED_EDGE('',*,*,#13901,.T.);
#19056=ORIENTED_EDGE('',*,*,#13904,.T.);
#19057=ORIENTED_EDGE('',*,*,#13906,.T.);
#19058=ORIENTED_EDGE('',*,*,#13910,.T.);
#19059=ORIENTED_EDGE('',*,*,#13913,.T.);
#19060=ORIENTED_EDGE('',*,*,#13916,.T.);
#19061=ORIENTED_EDGE('',*,*,#13918,.T.);
#19062=ORIENTED_EDGE('',*,*,#13922,.T.);
#19063=ORIENTED_EDGE('',*,*,#13925,.T.);
#19064=ORIENTED_EDGE('',*,*,#13928,.T.);
#19065=ORIENTED_EDGE('',*,*,#13932,.T.);
#19066=ORIENTED_EDGE('',*,*,#13935,.T.);
#19067=ORIENTED_EDGE('',*,*,#13938,.T.);
#19068=ORIENTED_EDGE('',*,*,#13939,.F.);
#19069=ORIENTED_EDGE('',*,*,#13881,.T.);
#19070=ORIENTED_EDGE('',*,*,#13855,.T.);
#19071=ORIENTED_EDGE('',*,*,#13859,.T.);
#19072=ORIENTED_EDGE('',*,*,#13862,.T.);
#19073=ORIENTED_EDGE('',*,*,#13865,.T.);
#23808=ADVANCED_FACE('',(#3055),#1504,.T.);
#23809=ADVANCED_FACE('',(#3056),#1505,.T.);
#23810=ADVANCED_FACE('',(#3057),#1506,.T.);
#23811=ADVANCED_FACE('',(#3058),#1507,.T.);
#23812=ADVANCED_FACE('',(#3059),#1508,.T.);
#23813=ADVANCED_FACE('',(#3060),#1509,.T.);
#23814=ADVANCED_FACE('',(#3061),#1510,.T.);
#23815=ADVANCED_FACE('',(#3062),#1511,.T.);
#23816=ADVANCED_FACE('',(#3063),#1512,.T.);
#23817=ADVANCED_FACE('',(#3064),#1513,.T.);
#23818=ADVANCED_FACE('',(#3065),#2187,.T.);
#23819=ADVANCED_FACE('',(#3066),#1514,.T.);
#23820=ADVANCED_FACE('',(#3067),#1515,.T.);
#23821=ADVANCED_FACE('',(#3068),#1516,.T.);
#23822=ADVANCED_FACE('',(#3069),#1517,.T.);
#23823=ADVANCED_FACE('',(#3070),#1518,.T.);
#23824=ADVANCED_FACE('',(#3071),#1519,.T.);
#23825=ADVANCED_FACE('',(#3072),#1520,.T.);
#23826=ADVANCED_FACE('',(#3073),#1521,.T.);
#23827=ADVANCED_FACE('',(#3074),#1522,.T.);
#23828=ADVANCED_FACE('',(#3075),#1523,.T.);
#23829=ADVANCED_FACE('',(#3076),#1524,.T.);
#23830=ADVANCED_FACE('',(#3077),#1525,.T.);
#23831=ADVANCED_FACE('',(#3078),#1526,.T.);
#23832=ADVANCED_FACE('',(#3079),#1527,.T.);
#23833=ADVANCED_FACE('',(#3080),#1528,.T.);
#23834=ADVANCED_FACE('',(#3081),#1529,.T.);
#23835=ADVANCED_FACE('',(#3082),#1530,.T.);
#23836=ADVANCED_FACE('',(#3083),#1531,.T.);
#23837=ADVANCED_FACE('',(#3084),#1532,.T.);
#23838=ADVANCED_FACE('',(#3085),#1533,.T.);
#23839=ADVANCED_FACE('',(#3086),#1534,.T.);
#23840=ADVANCED_FACE('',(#3087),#2188,.F.);
#23841=ADVANCED_FACE('',(#3088),#2189,.F.);
#23842=ADVANCED_FACE('',(#3089),#2190,.F.);
#23843=ADVANCED_FACE('',(#3090),#2191,.F.);
#23844=ADVANCED_FACE('',(#3091,#1244,#1245,#1246,#1247),#1535,.T.);
#23845=ADVANCED_FACE('',(#3092),#2192,.T.);
#23846=ADVANCED_FACE('',(#3093,#1248,#1249,#1250,#1251,#1252,#1253,#1254,
#1255,#1256,#1257,#1258),#1536,.T.);
#24541=CLOSED_SHELL('',(#23808,#23809,#23810,#23811,#23812,#23813,#23814,
#23815,#23816,#23817,#23818,#23819,#23820,#23821,#23822,#23823,#23824,#23825,
#23826,#23827,#23828,#23829,#23830,#23831,#23832,#23833,#23834,#23835,#23836,
#23837,#23838,#23839,#23840,#23841,#23842,#23843,#23844,#23845,#23846));
#26099=AXIS2_PLACEMENT_3D('',#37558,#30661,#30662);
#26100=AXIS2_PLACEMENT_3D('',#37559,#30663,#30664);
#26101=AXIS2_PLACEMENT_3D('',#37568,#30669,#30670);
#26102=AXIS2_PLACEMENT_3D('',#37574,#30674,#30675);
#26103=AXIS2_PLACEMENT_3D('',#37580,#30679,#30680);
#26104=AXIS2_PLACEMENT_3D('',#37583,#30683,#30684);
#26105=AXIS2_PLACEMENT_3D('',#37584,#30685,#30686);
#26106=AXIS2_PLACEMENT_3D('',#37593,#30691,#30692);
#26107=AXIS2_PLACEMENT_3D('',#37599,#30696,#30697);
#26108=AXIS2_PLACEMENT_3D('',#37605,#30701,#30702);
#26109=AXIS2_PLACEMENT_3D('',#37608,#30705,#30706);
#26110=AXIS2_PLACEMENT_3D('',#37609,#30707,#30708);
#26111=AXIS2_PLACEMENT_3D('',#37611,#30709,#30710);
#26112=AXIS2_PLACEMENT_3D('',#37614,#30712,#30713);
#26113=AXIS2_PLACEMENT_3D('',#37615,#30714,#30715);
#26114=AXIS2_PLACEMENT_3D('',#37616,#30716,#30717);
#26115=AXIS2_PLACEMENT_3D('',#37625,#30722,#30723);
#26116=AXIS2_PLACEMENT_3D('',#37631,#30727,#30728);
#26117=AXIS2_PLACEMENT_3D('',#37637,#30732,#30733);
#26118=AXIS2_PLACEMENT_3D('',#37640,#30736,#30737);
#26119=AXIS2_PLACEMENT_3D('',#37641,#30738,#30739);
#26120=AXIS2_PLACEMENT_3D('',#37650,#30744,#30745);
#26121=AXIS2_PLACEMENT_3D('',#37656,#30749,#30750);
#26122=AXIS2_PLACEMENT_3D('',#37662,#30754,#30755);
#26123=AXIS2_PLACEMENT_3D('',#37665,#30758,#30759);
#26124=AXIS2_PLACEMENT_3D('',#37666,#30760,#30761);
#26125=AXIS2_PLACEMENT_3D('',#37675,#30766,#30767);
#26126=AXIS2_PLACEMENT_3D('',#37681,#30771,#30772);
#26127=AXIS2_PLACEMENT_3D('',#37687,#30776,#30777);
#26128=AXIS2_PLACEMENT_3D('',#37690,#30780,#30781);
#26129=AXIS2_PLACEMENT_3D('',#37691,#30782,#30783);
#26130=AXIS2_PLACEMENT_3D('',#37700,#30788,#30789);
#26131=AXIS2_PLACEMENT_3D('',#37706,#30793,#30794);
#26132=AXIS2_PLACEMENT_3D('',#37712,#30798,#30799);
#26133=AXIS2_PLACEMENT_3D('',#37715,#30802,#30803);
#26134=AXIS2_PLACEMENT_3D('',#37716,#30804,#30805);
#26135=AXIS2_PLACEMENT_3D('',#37718,#30806,#30807);
#26136=AXIS2_PLACEMENT_3D('',#37721,#30809,#30810);
#26137=AXIS2_PLACEMENT_3D('',#37722,#30811,#30812);
#26138=AXIS2_PLACEMENT_3D('',#37724,#30813,#30814);
#26139=AXIS2_PLACEMENT_3D('',#37727,#30816,#30817);
#26140=AXIS2_PLACEMENT_3D('',#37728,#30818,#30819);
#26141=AXIS2_PLACEMENT_3D('',#37730,#30820,#30821);
#26142=AXIS2_PLACEMENT_3D('',#37733,#30823,#30824);
#26143=AXIS2_PLACEMENT_3D('',#37734,#30825,#30826);
#26144=AXIS2_PLACEMENT_3D('',#37736,#30827,#30828);
#26145=AXIS2_PLACEMENT_3D('',#37739,#30830,#30831);
#26146=AXIS2_PLACEMENT_3D('',#37740,#30832,#30833);
#26147=AXIS2_PLACEMENT_3D('',#37742,#30834,#30835);
#26148=AXIS2_PLACEMENT_3D('',#37743,#30836,#30837);
#26149=AXIS2_PLACEMENT_3D('',#37745,#30838,#30839);
#26150=AXIS2_PLACEMENT_3D('',#37747,#30841,#30842);
#30661=DIRECTION('axis',(0.,0.,1.));
#30662=DIRECTION('refdir',(1.,0.,0.));
#30663=DIRECTION('center_axis',(0.,1.,0.));
#30664=DIRECTION('ref_axis',(-1.,0.,0.));
#30665=DIRECTION('',(1.,0.,0.));
#30666=DIRECTION('',(0.,0.,1.));
#30667=DIRECTION('',(-1.,0.,0.));
#30668=DIRECTION('',(0.,0.,1.));
#30669=DIRECTION('center_axis',(1.,0.,0.));
#30670=DIRECTION('ref_axis',(0.,1.,0.));
#30671=DIRECTION('',(0.,-1.,0.));
#30672=DIRECTION('',(0.,1.,0.));
#30673=DIRECTION('',(0.,0.,1.));
#30674=DIRECTION('center_axis',(0.,-1.,0.));
#30675=DIRECTION('ref_axis',(1.,0.,0.));
#30676=DIRECTION('',(-1.,0.,0.));
#30677=DIRECTION('',(1.,0.,0.));
#30678=DIRECTION('',(0.,0.,1.));
#30679=DIRECTION('center_axis',(-1.,0.,0.));
#30680=DIRECTION('ref_axis',(0.,-1.,0.));
#30681=DIRECTION('',(0.,1.,0.));
#30682=DIRECTION('',(0.,-1.,0.));
#30683=DIRECTION('center_axis',(0.,0.,1.));
#30684=DIRECTION('ref_axis',(1.,0.,0.));
#30685=DIRECTION('center_axis',(0.,1.,0.));
#30686=DIRECTION('ref_axis',(-1.,0.,0.));
#30687=DIRECTION('',(1.,0.,0.));
#30688=DIRECTION('',(0.,0.,1.));
#30689=DIRECTION('',(-1.,0.,0.));
#30690=DIRECTION('',(0.,0.,1.));
#30691=DIRECTION('center_axis',(1.,0.,0.));
#30692=DIRECTION('ref_axis',(0.,1.,0.));
#30693=DIRECTION('',(0.,-1.,0.));
#30694=DIRECTION('',(0.,1.,0.));
#30695=DIRECTION('',(0.,0.,1.));
#30696=DIRECTION('center_axis',(0.,-1.,0.));
#30697=DIRECTION('ref_axis',(1.,0.,0.));
#30698=DIRECTION('',(-1.,0.,0.));
#30699=DIRECTION('',(1.,0.,0.));
#30700=DIRECTION('',(0.,0.,1.));
#30701=DIRECTION('center_axis',(-1.,0.,0.));
#30702=DIRECTION('ref_axis',(0.,-1.,0.));
#30703=DIRECTION('',(0.,1.,0.));
#30704=DIRECTION('',(0.,-1.,0.));
#30705=DIRECTION('center_axis',(0.,0.,1.));
#30706=DIRECTION('ref_axis',(1.,0.,0.));
#30707=DIRECTION('center_axis',(0.,0.,1.));
#30708=DIRECTION('ref_axis',(1.,0.,0.));
#30709=DIRECTION('center_axis',(0.,0.,1.));
#30710=DIRECTION('ref_axis',(1.,0.,0.));
#30711=DIRECTION('',(0.,0.,-1.));
#30712=DIRECTION('center_axis',(0.,0.,-1.));
#30713=DIRECTION('ref_axis',(1.,0.,0.));
#30714=DIRECTION('center_axis',(0.,0.,1.));
#30715=DIRECTION('ref_axis',(1.,0.,0.));
#30716=DIRECTION('center_axis',(0.,1.,0.));
#30717=DIRECTION('ref_axis',(-1.,0.,0.));
#30718=DIRECTION('',(1.,0.,0.));
#30719=DIRECTION('',(0.,0.,1.));
#30720=DIRECTION('',(-1.,0.,0.));
#30721=DIRECTION('',(0.,0.,1.));
#30722=DIRECTION('center_axis',(1.,0.,0.));
#30723=DIRECTION('ref_axis',(0.,1.,0.));
#30724=DIRECTION('',(0.,-1.,0.));
#30725=DIRECTION('',(0.,1.,0.));
#30726=DIRECTION('',(0.,0.,1.));
#30727=DIRECTION('center_axis',(0.,-1.,0.));
#30728=DIRECTION('ref_axis',(1.,0.,0.));
#30729=DIRECTION('',(-1.,0.,0.));
#30730=DIRECTION('',(1.,0.,0.));
#30731=DIRECTION('',(0.,0.,1.));
#30732=DIRECTION('center_axis',(-1.,0.,0.));
#30733=DIRECTION('ref_axis',(0.,-1.,0.));
#30734=DIRECTION('',(0.,1.,0.));
#30735=DIRECTION('',(0.,-1.,0.));
#30736=DIRECTION('center_axis',(0.,0.,1.));
#30737=DIRECTION('ref_axis',(1.,0.,0.));
#30738=DIRECTION('center_axis',(0.,1.,0.));
#30739=DIRECTION('ref_axis',(-1.,0.,0.));
#30740=DIRECTION('',(1.,0.,0.));
#30741=DIRECTION('',(0.,0.,1.));
#30742=DIRECTION('',(-1.,0.,0.));
#30743=DIRECTION('',(0.,0.,1.));
#30744=DIRECTION('center_axis',(1.,0.,0.));
#30745=DIRECTION('ref_axis',(0.,1.,0.));
#30746=DIRECTION('',(0.,-1.,0.));
#30747=DIRECTION('',(0.,1.,0.));
#30748=DIRECTION('',(0.,0.,1.));
#30749=DIRECTION('center_axis',(0.,-1.,0.));
#30750=DIRECTION('ref_axis',(1.,0.,0.));
#30751=DIRECTION('',(-1.,0.,0.));
#30752=DIRECTION('',(1.,0.,0.));
#30753=DIRECTION('',(0.,0.,1.));
#30754=DIRECTION('center_axis',(-1.,0.,0.));
#30755=DIRECTION('ref_axis',(0.,-1.,0.));
#30756=DIRECTION('',(0.,1.,0.));
#30757=DIRECTION('',(0.,-1.,0.));
#30758=DIRECTION('center_axis',(0.,0.,1.));
#30759=DIRECTION('ref_axis',(1.,0.,0.));
#30760=DIRECTION('center_axis',(0.,1.,0.));
#30761=DIRECTION('ref_axis',(-1.,0.,0.));
#30762=DIRECTION('',(1.,0.,0.));
#30763=DIRECTION('',(0.,0.,1.));
#30764=DIRECTION('',(-1.,0.,0.));
#30765=DIRECTION('',(0.,0.,1.));
#30766=DIRECTION('center_axis',(1.,0.,0.));
#30767=DIRECTION('ref_axis',(0.,1.,0.));
#30768=DIRECTION('',(0.,-1.,0.));
#30769=DIRECTION('',(0.,1.,0.));
#30770=DIRECTION('',(0.,0.,1.));
#30771=DIRECTION('center_axis',(0.,-1.,0.));
#30772=DIRECTION('ref_axis',(1.,0.,0.));
#30773=DIRECTION('',(-1.,0.,0.));
#30774=DIRECTION('',(1.,0.,0.));
#30775=DIRECTION('',(0.,0.,1.));
#30776=DIRECTION('center_axis',(-1.,0.,0.));
#30777=DIRECTION('ref_axis',(0.,-1.,0.));
#30778=DIRECTION('',(0.,1.,0.));
#30779=DIRECTION('',(0.,-1.,0.));
#30780=DIRECTION('center_axis',(0.,0.,1.));
#30781=DIRECTION('ref_axis',(1.,0.,0.));
#30782=DIRECTION('center_axis',(0.,1.,0.));
#30783=DIRECTION('ref_axis',(-1.,0.,0.));
#30784=DIRECTION('',(1.,0.,0.));
#30785=DIRECTION('',(0.,0.,1.));
#30786=DIRECTION('',(-1.,0.,0.));
#30787=DIRECTION('',(0.,0.,1.));
#30788=DIRECTION('center_axis',(1.,0.,0.));
#30789=DIRECTION('ref_axis',(0.,1.,0.));
#30790=DIRECTION('',(0.,-1.,0.));
#30791=DIRECTION('',(0.,1.,0.));
#30792=DIRECTION('',(0.,0.,1.));
#30793=DIRECTION('center_axis',(0.,-1.,0.));
#30794=DIRECTION('ref_axis',(1.,0.,0.));
#30795=DIRECTION('',(-1.,0.,0.));
#30796=DIRECTION('',(1.,0.,0.));
#30797=DIRECTION('',(0.,0.,1.));
#30798=DIRECTION('center_axis',(-1.,0.,0.));
#30799=DIRECTION('ref_axis',(0.,-1.,0.));
#30800=DIRECTION('',(0.,1.,0.));
#30801=DIRECTION('',(0.,-1.,0.));
#30802=DIRECTION('center_axis',(0.,0.,1.));
#30803=DIRECTION('ref_axis',(1.,0.,0.));
#30804=DIRECTION('center_axis',(0.,0.,1.));
#30805=DIRECTION('ref_axis',(1.,0.,0.));
#30806=DIRECTION('center_axis',(0.,0.,1.));
#30807=DIRECTION('ref_axis',(1.,0.,0.));
#30808=DIRECTION('',(0.,0.,1.));
#30809=DIRECTION('center_axis',(0.,0.,-1.));
#30810=DIRECTION('ref_axis',(1.,0.,0.));
#30811=DIRECTION('center_axis',(0.,0.,1.));
#30812=DIRECTION('ref_axis',(1.,0.,0.));
#30813=DIRECTION('center_axis',(0.,0.,1.));
#30814=DIRECTION('ref_axis',(1.,0.,0.));
#30815=DIRECTION('',(0.,0.,1.));
#30816=DIRECTION('center_axis',(0.,0.,-1.));
#30817=DIRECTION('ref_axis',(1.,0.,0.));
#30818=DIRECTION('center_axis',(0.,0.,1.));
#30819=DIRECTION('ref_axis',(1.,0.,0.));
#30820=DIRECTION('center_axis',(0.,0.,1.));
#30821=DIRECTION('ref_axis',(1.,0.,0.));
#30822=DIRECTION('',(0.,0.,1.));
#30823=DIRECTION('center_axis',(0.,0.,-1.));
#30824=DIRECTION('ref_axis',(1.,0.,0.));
#30825=DIRECTION('center_axis',(0.,0.,1.));
#30826=DIRECTION('ref_axis',(1.,0.,0.));
#30827=DIRECTION('center_axis',(0.,0.,1.));
#30828=DIRECTION('ref_axis',(1.,0.,0.));
#30829=DIRECTION('',(0.,0.,-1.));
#30830=DIRECTION('center_axis',(0.,0.,1.));
#30831=DIRECTION('ref_axis',(1.,0.,0.));
#30832=DIRECTION('center_axis',(0.,0.,-1.));
#30833=DIRECTION('ref_axis',(-1.,0.,0.));
#30834=DIRECTION('center_axis',(0.,0.,1.));
#30835=DIRECTION('ref_axis',(1.,0.,0.));
#30836=DIRECTION('center_axis',(0.,0.,1.));
#30837=DIRECTION('ref_axis',(1.,0.,0.));
#30838=DIRECTION('center_axis',(0.,0.,1.));
#30839=DIRECTION('ref_axis',(1.,0.,0.));
#30840=DIRECTION('',(0.,0.,-1.));
#30841=DIRECTION('center_axis',(0.,0.,1.));
#30842=DIRECTION('ref_axis',(1.,0.,0.));
#37558=CARTESIAN_POINT('',(0.,0.,0.));
#37559=CARTESIAN_POINT('Origin',(2.4,0.9,3.16));
#37560=CARTESIAN_POINT('',(1.8,0.9,3.16));
#37561=CARTESIAN_POINT('',(2.4,0.9,3.16));
#37562=CARTESIAN_POINT('',(1.6,0.9,3.16));
#37563=CARTESIAN_POINT('',(1.8,0.9,3.46));
#37564=CARTESIAN_POINT('',(1.8,0.9,3.16));
#37565=CARTESIAN_POINT('',(2.4,0.9,3.46));
#37566=CARTESIAN_POINT('',(2.4,0.9,3.46));
#37567=CARTESIAN_POINT('',(2.4,0.9,3.16));
#37568=CARTESIAN_POINT('Origin',(2.4,0.6,3.16));
#37569=CARTESIAN_POINT('',(2.4,0.6,3.16));
#37570=CARTESIAN_POINT('',(2.4,0.3,3.16));
#37571=CARTESIAN_POINT('',(2.4,0.6,3.46));
#37572=CARTESIAN_POINT('',(2.4,0.6,3.46));
#37573=CARTESIAN_POINT('',(2.4,0.6,3.16));
#37574=CARTESIAN_POINT('Origin',(1.8,0.6,3.16));
#37575=CARTESIAN_POINT('',(1.8,0.6,3.16));
#37576=CARTESIAN_POINT('',(1.3,0.6,3.16));
#37577=CARTESIAN_POINT('',(1.8,0.6,3.46));
#37578=CARTESIAN_POINT('',(1.8,0.6,3.46));
#37579=CARTESIAN_POINT('',(1.8,0.6,3.16));
#37580=CARTESIAN_POINT('Origin',(1.8,0.9,3.16));
#37581=CARTESIAN_POINT('',(1.8,0.45,3.16));
#37582=CARTESIAN_POINT('',(1.8,0.9,3.46));
#37583=CARTESIAN_POINT('Origin',(2.1,0.75,3.46));
#37584=CARTESIAN_POINT('Origin',(0.3,-2.6,3.16));
#37585=CARTESIAN_POINT('',(-0.9,-2.6,3.16));
#37586=CARTESIAN_POINT('',(0.3,-2.6,3.16));
#37587=CARTESIAN_POINT('',(0.55,-2.6,3.16));
#37588=CARTESIAN_POINT('',(-0.9,-2.6,3.76));
#37589=CARTESIAN_POINT('',(-0.9,-2.6,3.16));
#37590=CARTESIAN_POINT('',(0.3,-2.6,3.76));
#37591=CARTESIAN_POINT('',(0.3,-2.6,3.76));
#37592=CARTESIAN_POINT('',(0.3,-2.6,3.16));
#37593=CARTESIAN_POINT('Origin',(0.3,-3.2,3.16));
#37594=CARTESIAN_POINT('',(0.3,-3.2,3.16));
#37595=CARTESIAN_POINT('',(0.3,-1.6,3.16));
#37596=CARTESIAN_POINT('',(0.3,-3.2,3.76));
#37597=CARTESIAN_POINT('',(0.3,-3.2,3.76));
#37598=CARTESIAN_POINT('',(0.3,-3.2,3.16));
#37599=CARTESIAN_POINT('Origin',(-0.9,-3.2,3.16));
#37600=CARTESIAN_POINT('',(-0.9,-3.2,3.16));
#37601=CARTESIAN_POINT('',(-0.0500000000000001,-3.2,3.16));
#37602=CARTESIAN_POINT('',(-0.9,-3.2,3.76));
#37603=CARTESIAN_POINT('',(-0.9,-3.2,3.76));
#37604=CARTESIAN_POINT('',(-0.9,-3.2,3.16));
#37605=CARTESIAN_POINT('Origin',(-0.9,-2.6,3.16));
#37606=CARTESIAN_POINT('',(-0.9,-1.3,3.16));
#37607=CARTESIAN_POINT('',(-0.9,-2.6,3.76));
#37608=CARTESIAN_POINT('Origin',(-0.3,-2.9,3.76));
#37609=CARTESIAN_POINT('Origin',(2.,-1.,3.16));
#37610=CARTESIAN_POINT('',(1.7,-1.,3.86));
#37611=CARTESIAN_POINT('Origin',(2.,-1.,3.86));
#37612=CARTESIAN_POINT('',(1.7,-1.,3.16));
#37613=CARTESIAN_POINT('',(1.7,-1.,3.16));
#37614=CARTESIAN_POINT('Origin',(2.,-1.,3.16));
#37615=CARTESIAN_POINT('Origin',(2.,-1.,3.86));
#37616=CARTESIAN_POINT('Origin',(-0.5,2.4,3.16));
#37617=CARTESIAN_POINT('',(-1.,2.4,3.16));
#37618=CARTESIAN_POINT('',(-0.5,2.4,3.16));
#37619=CARTESIAN_POINT('',(0.15,2.4,3.16));
#37620=CARTESIAN_POINT('',(-1.,2.4,3.31));
#37621=CARTESIAN_POINT('',(-1.,2.4,3.16));
#37622=CARTESIAN_POINT('',(-0.5,2.4,3.31));
#37623=CARTESIAN_POINT('',(-0.5,2.4,3.31));
#37624=CARTESIAN_POINT('',(-0.5,2.4,3.16));
#37625=CARTESIAN_POINT('Origin',(-0.5,1.8,3.16));
#37626=CARTESIAN_POINT('',(-0.5,1.8,3.16));
#37627=CARTESIAN_POINT('',(-0.5,0.9,3.16));
#37628=CARTESIAN_POINT('',(-0.5,1.8,3.31));
#37629=CARTESIAN_POINT('',(-0.5,1.8,3.31));
#37630=CARTESIAN_POINT('',(-0.5,1.8,3.16));
#37631=CARTESIAN_POINT('Origin',(-1.,1.8,3.16));
#37632=CARTESIAN_POINT('',(-1.,1.8,3.16));
#37633=CARTESIAN_POINT('',(-0.1,1.8,3.16));
#37634=CARTESIAN_POINT('',(-1.,1.8,3.31));
#37635=CARTESIAN_POINT('',(-1.,1.8,3.31));
#37636=CARTESIAN_POINT('',(-1.,1.8,3.16));
#37637=CARTESIAN_POINT('Origin',(-1.,2.4,3.16));
#37638=CARTESIAN_POINT('',(-1.,1.2,3.16));
#37639=CARTESIAN_POINT('',(-1.,2.4,3.31));
#37640=CARTESIAN_POINT('Origin',(-0.75,2.1,3.31));
#37641=CARTESIAN_POINT('Origin',(-1.3,0.3,3.16));
#37642=CARTESIAN_POINT('',(-1.8,0.3,3.16));
#37643=CARTESIAN_POINT('',(-1.3,0.3,3.16));
#37644=CARTESIAN_POINT('',(-0.25,0.3,3.16));
#37645=CARTESIAN_POINT('',(-1.8,0.3,3.31));
#37646=CARTESIAN_POINT('',(-1.8,0.3,3.16));
#37647=CARTESIAN_POINT('',(-1.3,0.3,3.31));
#37648=CARTESIAN_POINT('',(-1.3,0.3,3.31));
#37649=CARTESIAN_POINT('',(-1.3,0.3,3.16));
#37650=CARTESIAN_POINT('Origin',(-1.3,-0.3,3.16));
#37651=CARTESIAN_POINT('',(-1.3,-0.3,3.16));
#37652=CARTESIAN_POINT('',(-1.3,-0.15,3.16));
#37653=CARTESIAN_POINT('',(-1.3,-0.3,3.31));
#37654=CARTESIAN_POINT('',(-1.3,-0.3,3.31));
#37655=CARTESIAN_POINT('',(-1.3,-0.3,3.16));
#37656=CARTESIAN_POINT('Origin',(-1.8,-0.3,3.16));
#37657=CARTESIAN_POINT('',(-1.8,-0.3,3.16));
#37658=CARTESIAN_POINT('',(-0.5,-0.3,3.16));
#37659=CARTESIAN_POINT('',(-1.8,-0.3,3.31));
#37660=CARTESIAN_POINT('',(-1.8,-0.3,3.31));
#37661=CARTESIAN_POINT('',(-1.8,-0.3,3.16));
#37662=CARTESIAN_POINT('Origin',(-1.8,0.3,3.16));
#37663=CARTESIAN_POINT('',(-1.8,0.15,3.16));
#37664=CARTESIAN_POINT('',(-1.8,0.3,3.31));
#37665=CARTESIAN_POINT('Origin',(-1.55,0.,3.31));
#37666=CARTESIAN_POINT('Origin',(-1.3,1.2,3.16));
#37667=CARTESIAN_POINT('',(-1.8,1.2,3.16));
#37668=CARTESIAN_POINT('',(-1.3,1.2,3.16));
#37669=CARTESIAN_POINT('',(-0.25,1.2,3.16));
#37670=CARTESIAN_POINT('',(-1.8,1.2,3.31));
#37671=CARTESIAN_POINT('',(-1.8,1.2,3.16));
#37672=CARTESIAN_POINT('',(-1.3,1.2,3.31));
#37673=CARTESIAN_POINT('',(-1.3,1.2,3.31));
#37674=CARTESIAN_POINT('',(-1.3,1.2,3.16));
#37675=CARTESIAN_POINT('Origin',(-1.3,0.6,3.16));
#37676=CARTESIAN_POINT('',(-1.3,0.6,3.16));
#37677=CARTESIAN_POINT('',(-1.3,0.3,3.16));
#37678=CARTESIAN_POINT('',(-1.3,0.6,3.31));
#37679=CARTESIAN_POINT('',(-1.3,0.6,3.31));
#37680=CARTESIAN_POINT('',(-1.3,0.6,3.16));
#37681=CARTESIAN_POINT('Origin',(-1.8,0.6,3.16));
#37682=CARTESIAN_POINT('',(-1.8,0.6,3.16));
#37683=CARTESIAN_POINT('',(-0.5,0.6,3.16));
#37684=CARTESIAN_POINT('',(-1.8,0.6,3.31));
#37685=CARTESIAN_POINT('',(-1.8,0.6,3.31));
#37686=CARTESIAN_POINT('',(-1.8,0.6,3.16));
#37687=CARTESIAN_POINT('Origin',(-1.8,1.2,3.16));
#37688=CARTESIAN_POINT('',(-1.8,0.6,3.16));
#37689=CARTESIAN_POINT('',(-1.8,1.2,3.31));
#37690=CARTESIAN_POINT('Origin',(-1.55,0.9,3.31));
#37691=CARTESIAN_POINT('Origin',(1.6,1.6,3.16));
#37692=CARTESIAN_POINT('',(0.8,1.6,3.16));
#37693=CARTESIAN_POINT('',(1.6,1.6,3.16));
#37694=CARTESIAN_POINT('',(1.2,1.6,3.16));
#37695=CARTESIAN_POINT('',(0.8,1.6,3.28));
#37696=CARTESIAN_POINT('',(0.8,1.6,3.16));
#37697=CARTESIAN_POINT('',(1.6,1.6,3.28));
#37698=CARTESIAN_POINT('',(1.6,1.6,3.28));
#37699=CARTESIAN_POINT('',(1.6,1.6,3.16));
#37700=CARTESIAN_POINT('Origin',(1.6,0.8,3.16));
#37701=CARTESIAN_POINT('',(1.6,0.8,3.16));
#37702=CARTESIAN_POINT('',(1.6,0.4,3.16));
#37703=CARTESIAN_POINT('',(1.6,0.8,3.28));
#37704=CARTESIAN_POINT('',(1.6,0.8,3.28));
#37705=CARTESIAN_POINT('',(1.6,0.8,3.16));
#37706=CARTESIAN_POINT('Origin',(0.8,0.8,3.16));
#37707=CARTESIAN_POINT('',(0.8,0.8,3.16));
#37708=CARTESIAN_POINT('',(0.8,0.8,3.16));
#37709=CARTESIAN_POINT('',(0.8,0.8,3.28));
#37710=CARTESIAN_POINT('',(0.8,0.8,3.28));
#37711=CARTESIAN_POINT('',(0.8,0.8,3.16));
#37712=CARTESIAN_POINT('Origin',(0.8,1.6,3.16));
#37713=CARTESIAN_POINT('',(0.8,0.8,3.16));
#37714=CARTESIAN_POINT('',(0.8,1.6,3.28));
#37715=CARTESIAN_POINT('Origin',(1.2,1.2,3.28));
#37716=CARTESIAN_POINT('Origin',(2.94448637286709,-1.7,3.085));
#37717=CARTESIAN_POINT('',(2.80948637286709,-1.7,3.));
#37718=CARTESIAN_POINT('Origin',(2.94448637286709,-1.7,3.));
#37719=CARTESIAN_POINT('',(2.80948637286709,-1.7,3.16));
#37720=CARTESIAN_POINT('',(2.80948637286709,-1.7,3.085));
#37721=CARTESIAN_POINT('Origin',(2.94448637286709,-1.7,3.16));
#37722=CARTESIAN_POINT('Origin',(-2.94448637286709,-1.7,3.085));
#37723=CARTESIAN_POINT('',(-3.07948637286709,-1.7,3.));
#37724=CARTESIAN_POINT('Origin',(-2.94448637286709,-1.7,3.));
#37725=CARTESIAN_POINT('',(-3.07948637286709,-1.7,3.16));
#37726=CARTESIAN_POINT('',(-3.07948637286709,-1.7,3.085));
#37727=CARTESIAN_POINT('Origin',(-2.94448637286709,-1.7,3.16));
#37728=CARTESIAN_POINT('Origin',(2.0818995585505E-16,3.4,3.085));
#37729=CARTESIAN_POINT('',(-0.135,3.4,3.));
#37730=CARTESIAN_POINT('Origin',(2.0818995585505E-16,3.4,3.));
#37731=CARTESIAN_POINT('',(-0.135,3.4,3.16));
#37732=CARTESIAN_POINT('',(-0.135,3.4,3.085));
#37733=CARTESIAN_POINT('Origin',(2.0818995585505E-16,3.4,3.16));
#37734=CARTESIAN_POINT('Origin',(0.,0.,3.08));
#37735=CARTESIAN_POINT('',(-0.8,-9.79717439317883E-17,3.16));
#37736=CARTESIAN_POINT('Origin',(0.,0.,3.16));
#37737=CARTESIAN_POINT('',(-0.8,-9.79717439317883E-17,3.));
#37738=CARTESIAN_POINT('',(-0.8,-9.79717439317883E-17,3.08));
#37739=CARTESIAN_POINT('Origin',(0.,0.,3.));
#37740=CARTESIAN_POINT('Origin',(3.8,0.,3.));
#37741=CARTESIAN_POINT('',(-3.8,-4.65365783675994E-16,3.));
#37742=CARTESIAN_POINT('Origin',(0.,0.,3.));
#37743=CARTESIAN_POINT('Origin',(0.,0.,3.08));
#37744=CARTESIAN_POINT('',(-3.8,-4.65365783675994E-16,3.16));
#37745=CARTESIAN_POINT('Origin',(0.,0.,3.16));
#37746=CARTESIAN_POINT('',(-3.8,-4.65365783675994E-16,3.08));
#37747=CARTESIAN_POINT('Origin',(0.8,0.,3.16));
#54972=UNCERTAINTY_MEASURE_WITH_UNIT(LENGTH_MEASURE(0.001),#55003,
'DISTANCE_ACCURACY_VALUE',
'Maximum model space distance between geometric entities at asserted c
onnectivities');
#54980=UNCERTAINTY_MEASURE_WITH_UNIT(LENGTH_MEASURE(0.001),#55003,
'DISTANCE_ACCURACY_VALUE',
'Maximum model space distance between geometric entities at asserted c
onnectivities');
#54994=(
GEOMETRIC_REPRESENTATION_CONTEXT(3)
GLOBAL_UNCERTAINTY_ASSIGNED_CONTEXT((#54972))
GLOBAL_UNIT_ASSIGNED_CONTEXT((#55003,#55005,#55006))
REPRESENTATION_CONTEXT('','3D')
);
#55002=(
GEOMETRIC_REPRESENTATION_CONTEXT(3)
GLOBAL_UNCERTAINTY_ASSIGNED_CONTEXT((#54980))
GLOBAL_UNIT_ASSIGNED_CONTEXT((#55003,#55005,#55006))
REPRESENTATION_CONTEXT('','3D')
);
#55003=(
LENGTH_UNIT()
NAMED_UNIT(*)
SI_UNIT(.CENTI.,.METRE.)
);
#55005=(
NAMED_UNIT(*)
PLANE_ANGLE_UNIT()
SI_UNIT($,.RADIAN.)
);
#55006=(
NAMED_UNIT(*)
SI_UNIT($,.STERADIAN.)
SOLID_ANGLE_UNIT()
);
#55020=SHAPE_DEFINITION_REPRESENTATION(#55041,#55116);
#55041=PRODUCT_DEFINITION_SHAPE('',$,#55138);
#55116=SHAPE_REPRESENTATION('',(#26099),#54994);
#55124=PRODUCT_DEFINITION_CONTEXT('part definition',#55189,'design');
#55138=PRODUCT_DEFINITION('2026-10-18-23-36-38-410',
'13_Motor_Speed_Controller_Board_D76',#55159,#55124);
#55159=PRODUCT_DEFINITION_FORMATION('',$,#55204);
#55189=APPLICATION_CONTEXT(
'Core Data for Automotive Mechanical Design Process');
#55190=PRODUCT_CONTEXT('part definition',#55189,'mechanical');
#55204=PRODUCT('2026-10-18-23-36-38-410',
'13_Motor_Speed_Controller_Board_D76',$,(#55190));
#55373=COLOUR_RGB('Sky Blue',0.24,0.69,0.87);
#55374=FILL_AREA_STYLE_COLOUR('',#55373);
#55375=FILL_AREA_STYLE('',(#55374));
#55376=SURFACE_STYLE_FILL_AREA(#55375);
#55377=SURFACE_SIDE_STYLE('',(#55376));
#55378=SURFACE_STYLE_USAGE(.BOTH.,#55377);
#55379=PRESENTATION_STYLE_ASSIGNMENT((#55378));
ENDSEC;
END-ISO-10303-21;
